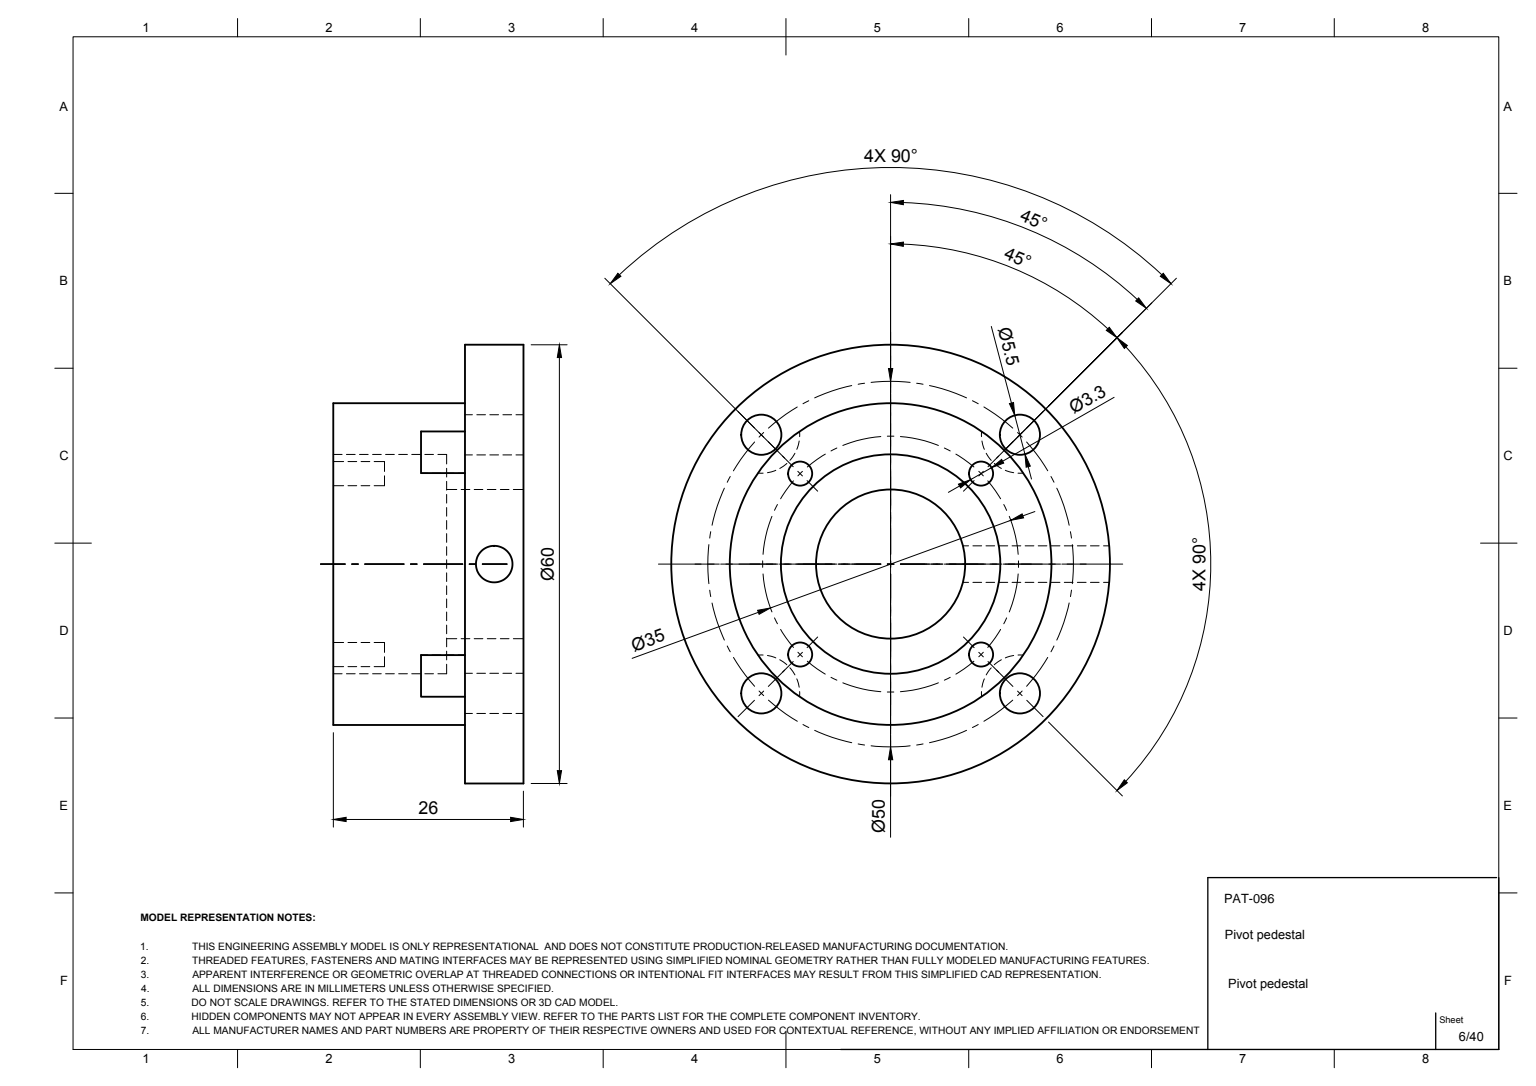
ISO-10303-21;
HEADER;
/* Generated by software containing ST-Developer
 * from STEP Tools, Inc. (www.steptools.com) 
 */

FILE_DESCRIPTION(
/* description */ ('PAT-096'),
/* implementation_level */ '2;1');

FILE_NAME(
/* name */ 'Pivot pedestal.step',
/* time_stamp */ '2026-10-29T17:03:14-07:00',
/* author */ (''),
/* organization */ (''),
/* preprocessor_version */ 'ST-DEVELOPER v20.2',
/* originating_system */ 'Autodesk Translation Framework v15.17.0.0',
/* authorisation */ '');

FILE_SCHEMA (('AUTOMOTIVE_DESIGN { 1 0 10303 214 3 1 1 }'));
ENDSEC;

DATA;
#10=MECHANICAL_DESIGN_GEOMETRIC_PRESENTATION_REPRESENTATION('',(#400),#10650);
#281=B_SPLINE_CURVE_WITH_KNOTS('',3,(#8659,#8660,#8661,#8662,#8663,#8664,
#8665,#8666,#8667,#8668),.UNSPECIFIED.,.F.,.F.,(4,2,2,2,4),(0.,0.0945941824764479,
0.189188364952896,0.283770357603024,0.378352350253152),.UNSPECIFIED.);
#282=B_SPLINE_CURVE_WITH_KNOTS('',3,(#8669,#8670,#8671,#8672,#8673,#8674,
#8675,#8676,#8677,#8678,#8679,#8680,#8681,#8682,#8683,#8684,#8685,#8686,
#8687,#8688,#8689,#8690,#8691,#8692,#8693,#8694),.UNSPECIFIED.,.F.,.F.,
(4,2,2,2,2,2,2,2,2,2,2,2,4),(0.378352350253152,0.47293434290328,0.567516335553408,
0.662110518029855,0.756704700506303,0.851298882982751,0.945893065459199,
1.04047505810933,1.13505705075946,1.22963904340958,1.32422103605971,1.41881521853616,
1.51340940101261),.UNSPECIFIED.);
#283=B_SPLINE_CURVE_WITH_KNOTS('',3,(#8698,#8699,#8700,#8701,#8702,#8703,
#8704,#8705,#8706,#8707,#8708,#8709,#8710,#8711,#8712,#8713,#8714,#8715,
#8716,#8717,#8718,#8719,#8720,#8721,#8722,#8723),.UNSPECIFIED.,.F.,.F.,
(4,2,2,2,2,2,2,2,2,2,2,2,4),(0.,0.0942186410044058,0.188437282008812,0.282655768798837,
0.376874255588861,0.471092742378886,0.565311229168911,0.659529870173317,
0.753748511177723,0.847967152182129,0.942185793186535,1.03640427997656,
1.13062276676658),.UNSPECIFIED.);
#284=B_SPLINE_CURVE_WITH_KNOTS('',3,(#8724,#8725,#8726,#8727,#8728,#8729,
#8730,#8731,#8732,#8733),.UNSPECIFIED.,.F.,.F.,(4,2,2,2,4),(1.13062276676658,
1.22484125355661,1.31905974034663,1.41327838135104,1.50749702235545),
 .UNSPECIFIED.);
#338=SHAPE_REPRESENTATION_RELATIONSHIP('SRR','None',#10798,#369);
#369=ADVANCED_BREP_SHAPE_REPRESENTATION('',(#438),#10616);
#400=STYLED_ITEM('',(#11078),#438);
#438=MANIFOLD_SOLID_BREP('Body1',#5534);
#490=FACE_BOUND('',#1192,.T.);
#491=FACE_BOUND('',#1193,.T.);
#492=FACE_BOUND('',#1194,.T.);
#493=FACE_BOUND('',#1195,.T.);
#494=FACE_BOUND('',#1196,.T.);
#495=FACE_BOUND('',#1203,.T.);
#496=FACE_BOUND('',#1205,.T.);
#497=FACE_BOUND('',#1207,.T.);
#498=FACE_BOUND('',#1209,.T.);
#499=FACE_BOUND('',#1210,.T.);
#500=FACE_BOUND('',#1211,.T.);
#501=FACE_BOUND('',#1212,.T.);
#502=FACE_BOUND('',#1213,.T.);
#503=FACE_BOUND('',#1215,.T.);
#504=FACE_BOUND('',#1216,.T.);
#505=FACE_BOUND('',#1217,.T.);
#506=FACE_BOUND('',#1218,.T.);
#507=FACE_BOUND('',#1219,.T.);
#629=PLANE('',#5977);
#630=PLANE('',#5981);
#631=PLANE('',#5985);
#632=PLANE('',#5989);
#633=PLANE('',#5990);
#634=PLANE('',#5998);
#635=PLANE('',#6003);
#636=PLANE('',#6008);
#637=PLANE('',#6017);
#638=PLANE('',#6034);
#639=PLANE('',#6040);
#640=PLANE('',#6041);
#820=FACE_OUTER_BOUND('',#1173,.T.);
#821=FACE_OUTER_BOUND('',#1174,.T.);
#822=FACE_OUTER_BOUND('',#1175,.T.);
#823=FACE_OUTER_BOUND('',#1176,.T.);
#824=FACE_OUTER_BOUND('',#1177,.T.);
#825=FACE_OUTER_BOUND('',#1178,.T.);
#826=FACE_OUTER_BOUND('',#1179,.T.);
#827=FACE_OUTER_BOUND('',#1180,.T.);
#828=FACE_OUTER_BOUND('',#1181,.T.);
#829=FACE_OUTER_BOUND('',#1182,.T.);
#830=FACE_OUTER_BOUND('',#1183,.T.);
#831=FACE_OUTER_BOUND('',#1184,.T.);
#832=FACE_OUTER_BOUND('',#1185,.T.);
#833=FACE_OUTER_BOUND('',#1186,.T.);
#834=FACE_OUTER_BOUND('',#1187,.T.);
#835=FACE_OUTER_BOUND('',#1188,.T.);
#836=FACE_OUTER_BOUND('',#1189,.T.);
#837=FACE_OUTER_BOUND('',#1190,.T.);
#838=FACE_OUTER_BOUND('',#1191,.T.);
#839=FACE_OUTER_BOUND('',#1197,.T.);
#840=FACE_OUTER_BOUND('',#1198,.T.);
#841=FACE_OUTER_BOUND('',#1199,.T.);
#842=FACE_OUTER_BOUND('',#1200,.T.);
#843=FACE_OUTER_BOUND('',#1201,.T.);
#844=FACE_OUTER_BOUND('',#1202,.T.);
#845=FACE_OUTER_BOUND('',#1204,.T.);
#846=FACE_OUTER_BOUND('',#1206,.T.);
#847=FACE_OUTER_BOUND('',#1208,.T.);
#848=FACE_OUTER_BOUND('',#1214,.T.);
#1173=EDGE_LOOP('',(#3847,#3848,#3849,#3850,#3851,#3852));
#1174=EDGE_LOOP('',(#3853,#3854,#3855,#3856));
#1175=EDGE_LOOP('',(#3857));
#1176=EDGE_LOOP('',(#3858,#3859,#3860,#3861));
#1177=EDGE_LOOP('',(#3862));
#1178=EDGE_LOOP('',(#3863,#3864,#3865,#3866));
#1179=EDGE_LOOP('',(#3867));
#1180=EDGE_LOOP('',(#3868,#3869,#3870,#3871));
#1181=EDGE_LOOP('',(#3872));
#1182=EDGE_LOOP('',(#3873,#3874));
#1183=EDGE_LOOP('',(#3875,#3876,#3877,#3878));
#1184=EDGE_LOOP('',(#3879,#3880,#3881,#3882));
#1185=EDGE_LOOP('',(#3883,#3884));
#1186=EDGE_LOOP('',(#3885,#3886,#3887,#3888));
#1187=EDGE_LOOP('',(#3889,#3890));
#1188=EDGE_LOOP('',(#3891,#3892,#3893,#3894));
#1189=EDGE_LOOP('',(#3895,#3896));
#1190=EDGE_LOOP('',(#3897,#3898,#3899,#3900,#3901,#3902,#3903,#3904,#3905,
#3906,#3907,#3908,#3909,#3910,#3911,#3912,#3913,#3914,#3915,#3916));
#1191=EDGE_LOOP('',(#3917));
#1192=EDGE_LOOP('',(#3918,#3919,#3920,#3921,#3922,#3923,#3924,#3925,#3926));
#1193=EDGE_LOOP('',(#3927));
#1194=EDGE_LOOP('',(#3928));
#1195=EDGE_LOOP('',(#3929));
#1196=EDGE_LOOP('',(#3930));
#1197=EDGE_LOOP('',(#3931,#3932,#3933,#3934));
#1198=EDGE_LOOP('',(#3935,#3936,#3937,#3938));
#1199=EDGE_LOOP('',(#3939,#3940,#3941,#3942));
#1200=EDGE_LOOP('',(#3943,#3944,#3945,#3946));
#1201=EDGE_LOOP('',(#3947,#3948,#3949,#3950));
#1202=EDGE_LOOP('',(#3951));
#1203=EDGE_LOOP('',(#3952));
#1204=EDGE_LOOP('',(#3953,#3954,#3955,#3956));
#1205=EDGE_LOOP('',(#3957,#3958));
#1206=EDGE_LOOP('',(#3959,#3960,#3961,#3962));
#1207=EDGE_LOOP('',(#3963,#3964));
#1208=EDGE_LOOP('',(#3965));
#1209=EDGE_LOOP('',(#3966));
#1210=EDGE_LOOP('',(#3967));
#1211=EDGE_LOOP('',(#3968));
#1212=EDGE_LOOP('',(#3969));
#1213=EDGE_LOOP('',(#3970));
#1214=EDGE_LOOP('',(#3971));
#1215=EDGE_LOOP('',(#3972));
#1216=EDGE_LOOP('',(#3973));
#1217=EDGE_LOOP('',(#3974));
#1218=EDGE_LOOP('',(#3975));
#1219=EDGE_LOOP('',(#3976));
#1644=LINE('',#8696,#1973);
#1645=LINE('',#8738,#1974);
#1646=LINE('',#8745,#1975);
#1647=LINE('',#8752,#1976);
#1648=LINE('',#8759,#1977);
#1649=LINE('',#8769,#1978);
#1650=LINE('',#8772,#1979);
#1651=LINE('',#8776,#1980);
#1652=LINE('',#8780,#1981);
#1653=LINE('',#8787,#1982);
#1654=LINE('',#8791,#1983);
#1655=LINE('',#8798,#1984);
#1656=LINE('',#8802,#1985);
#1657=LINE('',#8810,#1986);
#1658=LINE('',#8830,#1987);
#1659=LINE('',#8834,#1988);
#1660=LINE('',#8838,#1989);
#1661=LINE('',#8842,#1990);
#1662=LINE('',#8847,#1991);
#1663=LINE('',#8854,#1992);
#1664=LINE('',#8858,#1993);
#1973=VECTOR('',#6832,0.25);
#1974=VECTOR('',#6837,0.165);
#1975=VECTOR('',#6846,0.165);
#1976=VECTOR('',#6855,0.165);
#1977=VECTOR('',#6864,0.165);
#1978=VECTOR('',#6877,1.);
#1979=VECTOR('',#6880,1.);
#1980=VECTOR('',#6883,1.);
#1981=VECTOR('',#6886,1.);
#1982=VECTOR('',#6895,1.);
#1983=VECTOR('',#6898,1.);
#1984=VECTOR('',#6907,1.);
#1985=VECTOR('',#6910,1.);
#1986=VECTOR('',#6921,2.2);
#1987=VECTOR('',#6948,0.275);
#1988=VECTOR('',#6953,0.275);
#1989=VECTOR('',#6958,0.275);
#1990=VECTOR('',#6963,0.275);
#1991=VECTOR('',#6968,1.5);
#1992=VECTOR('',#6977,3.);
#1993=VECTOR('',#6982,1.02);
#2282=CIRCLE('',#5975,0.165);
#2283=CIRCLE('',#5976,0.165);
#2284=CIRCLE('',#5979,0.165);
#2285=CIRCLE('',#5980,0.165);
#2286=CIRCLE('',#5983,0.165);
#2287=CIRCLE('',#5984,0.165);
#2288=CIRCLE('',#5987,0.165);
#2289=CIRCLE('',#5988,0.165);
#2290=CIRCLE('',#5991,2.2);
#2291=CIRCLE('',#5992,0.525);
#2292=CIRCLE('',#5994,0.525);
#2293=CIRCLE('',#5996,0.525);
#2294=CIRCLE('',#5997,0.525);
#2295=CIRCLE('',#5999,2.2);
#2296=CIRCLE('',#6001,0.525);
#2297=CIRCLE('',#6002,0.525);
#2298=CIRCLE('',#6004,2.2);
#2299=CIRCLE('',#6006,0.525);
#2300=CIRCLE('',#6007,0.525);
#2301=CIRCLE('',#6009,2.2);
#2302=CIRCLE('',#6011,2.2);
#2303=CIRCLE('',#6012,2.2);
#2304=CIRCLE('',#6013,2.2);
#2305=CIRCLE('',#6014,2.2);
#2306=CIRCLE('',#6015,2.2);
#2307=CIRCLE('',#6016,2.2);
#2308=CIRCLE('',#6018,3.);
#2309=CIRCLE('',#6019,0.275);
#2310=CIRCLE('',#6020,0.275);
#2311=CIRCLE('',#6021,0.275);
#2312=CIRCLE('',#6022,0.275);
#2313=CIRCLE('',#6024,0.275);
#2314=CIRCLE('',#6026,0.275);
#2315=CIRCLE('',#6028,0.275);
#2316=CIRCLE('',#6030,0.275);
#2317=CIRCLE('',#6032,1.5);
#2318=CIRCLE('',#6033,1.5);
#2319=CIRCLE('',#6035,1.02);
#2320=CIRCLE('',#6037,3.);
#2321=CIRCLE('',#6039,1.02);
#2621=VERTEX_POINT('',#8657);
#2622=VERTEX_POINT('',#8658);
#2623=VERTEX_POINT('',#8695);
#2624=VERTEX_POINT('',#8697);
#2625=VERTEX_POINT('',#8735);
#2626=VERTEX_POINT('',#8737);
#2627=VERTEX_POINT('',#8742);
#2628=VERTEX_POINT('',#8744);
#2629=VERTEX_POINT('',#8749);
#2630=VERTEX_POINT('',#8751);
#2631=VERTEX_POINT('',#8756);
#2632=VERTEX_POINT('',#8758);
#2633=VERTEX_POINT('',#8763);
#2634=VERTEX_POINT('',#8764);
#2635=VERTEX_POINT('',#8768);
#2636=VERTEX_POINT('',#8770);
#2637=VERTEX_POINT('',#8774);
#2638=VERTEX_POINT('',#8775);
#2639=VERTEX_POINT('',#8777);
#2640=VERTEX_POINT('',#8779);
#2641=VERTEX_POINT('',#8785);
#2642=VERTEX_POINT('',#8786);
#2643=VERTEX_POINT('',#8788);
#2644=VERTEX_POINT('',#8790);
#2645=VERTEX_POINT('',#8796);
#2646=VERTEX_POINT('',#8797);
#2647=VERTEX_POINT('',#8799);
#2648=VERTEX_POINT('',#8801);
#2649=VERTEX_POINT('',#8807);
#2650=VERTEX_POINT('',#8809);
#2651=VERTEX_POINT('',#8817);
#2652=VERTEX_POINT('',#8819);
#2653=VERTEX_POINT('',#8821);
#2654=VERTEX_POINT('',#8823);
#2655=VERTEX_POINT('',#8825);
#2656=VERTEX_POINT('',#8828);
#2657=VERTEX_POINT('',#8832);
#2658=VERTEX_POINT('',#8836);
#2659=VERTEX_POINT('',#8840);
#2660=VERTEX_POINT('',#8844);
#2661=VERTEX_POINT('',#8846);
#2662=VERTEX_POINT('',#8850);
#2663=VERTEX_POINT('',#8853);
#2664=VERTEX_POINT('',#8857);
#3102=EDGE_CURVE('',#2621,#2622,#281,.T.);
#3103=EDGE_CURVE('',#2622,#2621,#282,.T.);
#3104=EDGE_CURVE('',#2622,#2623,#1644,.T.);
#3105=EDGE_CURVE('',#2624,#2623,#283,.T.);
#3106=EDGE_CURVE('',#2623,#2624,#284,.T.);
#3107=EDGE_CURVE('',#2625,#2625,#2282,.T.);
#3108=EDGE_CURVE('',#2625,#2626,#1645,.T.);
#3109=EDGE_CURVE('',#2626,#2626,#2283,.T.);
#3110=EDGE_CURVE('',#2627,#2627,#2284,.T.);
#3111=EDGE_CURVE('',#2627,#2628,#1646,.T.);
#3112=EDGE_CURVE('',#2628,#2628,#2285,.T.);
#3113=EDGE_CURVE('',#2629,#2629,#2286,.T.);
#3114=EDGE_CURVE('',#2629,#2630,#1647,.T.);
#3115=EDGE_CURVE('',#2630,#2630,#2287,.T.);
#3116=EDGE_CURVE('',#2631,#2631,#2288,.T.);
#3117=EDGE_CURVE('',#2631,#2632,#1648,.T.);
#3118=EDGE_CURVE('',#2632,#2632,#2289,.T.);
#3119=EDGE_CURVE('',#2633,#2634,#2290,.T.);
#3120=EDGE_CURVE('',#2634,#2633,#2291,.T.);
#3121=EDGE_CURVE('',#2635,#2633,#1649,.T.);
#3122=EDGE_CURVE('',#2636,#2635,#2292,.T.);
#3123=EDGE_CURVE('',#2634,#2636,#1650,.T.);
#3124=EDGE_CURVE('',#2637,#2638,#1651,.T.);
#3125=EDGE_CURVE('',#2637,#2639,#2293,.T.);
#3126=EDGE_CURVE('',#2640,#2639,#1652,.T.);
#3127=EDGE_CURVE('',#2638,#2640,#2294,.T.);
#3128=EDGE_CURVE('',#2639,#2637,#2295,.T.);
#3129=EDGE_CURVE('',#2641,#2642,#1653,.T.);
#3130=EDGE_CURVE('',#2641,#2643,#2296,.T.);
#3131=EDGE_CURVE('',#2644,#2643,#1654,.T.);
#3132=EDGE_CURVE('',#2642,#2644,#2297,.T.);
#3133=EDGE_CURVE('',#2643,#2641,#2298,.T.);
#3134=EDGE_CURVE('',#2645,#2646,#1655,.T.);
#3135=EDGE_CURVE('',#2645,#2647,#2299,.T.);
#3136=EDGE_CURVE('',#2648,#2647,#1656,.T.);
#3137=EDGE_CURVE('',#2646,#2648,#2300,.T.);
#3138=EDGE_CURVE('',#2647,#2645,#2301,.T.);
#3139=EDGE_CURVE('',#2649,#2649,#2302,.T.);
#3140=EDGE_CURVE('',#2649,#2650,#1657,.T.);
#3141=EDGE_CURVE('',#2650,#2635,#2303,.T.);
#3142=EDGE_CURVE('',#2636,#2648,#2304,.T.);
#3143=EDGE_CURVE('',#2646,#2644,#2305,.T.);
#3144=EDGE_CURVE('',#2642,#2640,#2306,.T.);
#3145=EDGE_CURVE('',#2638,#2650,#2307,.T.);
#3146=EDGE_CURVE('',#2651,#2651,#2308,.T.);
#3147=EDGE_CURVE('',#2652,#2652,#2309,.T.);
#3148=EDGE_CURVE('',#2653,#2653,#2310,.T.);
#3149=EDGE_CURVE('',#2654,#2654,#2311,.T.);
#3150=EDGE_CURVE('',#2655,#2655,#2312,.T.);
#3151=EDGE_CURVE('',#2656,#2656,#2313,.T.);
#3152=EDGE_CURVE('',#2656,#2652,#1658,.T.);
#3153=EDGE_CURVE('',#2657,#2657,#2314,.T.);
#3154=EDGE_CURVE('',#2657,#2655,#1659,.T.);
#3155=EDGE_CURVE('',#2658,#2658,#2315,.T.);
#3156=EDGE_CURVE('',#2658,#2653,#1660,.T.);
#3157=EDGE_CURVE('',#2659,#2659,#2316,.T.);
#3158=EDGE_CURVE('',#2659,#2654,#1661,.T.);
#3159=EDGE_CURVE('',#2660,#2660,#2317,.T.);
#3160=EDGE_CURVE('',#2660,#2661,#1662,.T.);
#3161=EDGE_CURVE('',#2661,#2661,#2318,.T.);
#3162=EDGE_CURVE('',#2662,#2662,#2319,.T.);
#3163=EDGE_CURVE('',#2651,#2663,#1663,.T.);
#3164=EDGE_CURVE('',#2663,#2663,#2320,.T.);
#3165=EDGE_CURVE('',#2662,#2664,#1664,.T.);
#3166=EDGE_CURVE('',#2664,#2664,#2321,.T.);
#3847=ORIENTED_EDGE('',*,*,#3102,.F.);
#3848=ORIENTED_EDGE('',*,*,#3103,.F.);
#3849=ORIENTED_EDGE('',*,*,#3104,.T.);
#3850=ORIENTED_EDGE('',*,*,#3105,.F.);
#3851=ORIENTED_EDGE('',*,*,#3106,.F.);
#3852=ORIENTED_EDGE('',*,*,#3104,.F.);
#3853=ORIENTED_EDGE('',*,*,#3107,.F.);
#3854=ORIENTED_EDGE('',*,*,#3108,.T.);
#3855=ORIENTED_EDGE('',*,*,#3109,.F.);
#3856=ORIENTED_EDGE('',*,*,#3108,.F.);
#3857=ORIENTED_EDGE('',*,*,#3107,.T.);
#3858=ORIENTED_EDGE('',*,*,#3110,.F.);
#3859=ORIENTED_EDGE('',*,*,#3111,.T.);
#3860=ORIENTED_EDGE('',*,*,#3112,.F.);
#3861=ORIENTED_EDGE('',*,*,#3111,.F.);
#3862=ORIENTED_EDGE('',*,*,#3110,.T.);
#3863=ORIENTED_EDGE('',*,*,#3113,.F.);
#3864=ORIENTED_EDGE('',*,*,#3114,.T.);
#3865=ORIENTED_EDGE('',*,*,#3115,.F.);
#3866=ORIENTED_EDGE('',*,*,#3114,.F.);
#3867=ORIENTED_EDGE('',*,*,#3113,.T.);
#3868=ORIENTED_EDGE('',*,*,#3116,.F.);
#3869=ORIENTED_EDGE('',*,*,#3117,.T.);
#3870=ORIENTED_EDGE('',*,*,#3118,.F.);
#3871=ORIENTED_EDGE('',*,*,#3117,.F.);
#3872=ORIENTED_EDGE('',*,*,#3116,.T.);
#3873=ORIENTED_EDGE('',*,*,#3119,.F.);
#3874=ORIENTED_EDGE('',*,*,#3120,.F.);
#3875=ORIENTED_EDGE('',*,*,#3121,.F.);
#3876=ORIENTED_EDGE('',*,*,#3122,.F.);
#3877=ORIENTED_EDGE('',*,*,#3123,.F.);
#3878=ORIENTED_EDGE('',*,*,#3120,.T.);
#3879=ORIENTED_EDGE('',*,*,#3124,.F.);
#3880=ORIENTED_EDGE('',*,*,#3125,.T.);
#3881=ORIENTED_EDGE('',*,*,#3126,.F.);
#3882=ORIENTED_EDGE('',*,*,#3127,.F.);
#3883=ORIENTED_EDGE('',*,*,#3128,.F.);
#3884=ORIENTED_EDGE('',*,*,#3125,.F.);
#3885=ORIENTED_EDGE('',*,*,#3129,.F.);
#3886=ORIENTED_EDGE('',*,*,#3130,.T.);
#3887=ORIENTED_EDGE('',*,*,#3131,.F.);
#3888=ORIENTED_EDGE('',*,*,#3132,.F.);
#3889=ORIENTED_EDGE('',*,*,#3133,.F.);
#3890=ORIENTED_EDGE('',*,*,#3130,.F.);
#3891=ORIENTED_EDGE('',*,*,#3134,.F.);
#3892=ORIENTED_EDGE('',*,*,#3135,.T.);
#3893=ORIENTED_EDGE('',*,*,#3136,.F.);
#3894=ORIENTED_EDGE('',*,*,#3137,.F.);
#3895=ORIENTED_EDGE('',*,*,#3138,.F.);
#3896=ORIENTED_EDGE('',*,*,#3135,.F.);
#3897=ORIENTED_EDGE('',*,*,#3139,.F.);
#3898=ORIENTED_EDGE('',*,*,#3140,.T.);
#3899=ORIENTED_EDGE('',*,*,#3141,.T.);
#3900=ORIENTED_EDGE('',*,*,#3121,.T.);
#3901=ORIENTED_EDGE('',*,*,#3119,.T.);
#3902=ORIENTED_EDGE('',*,*,#3123,.T.);
#3903=ORIENTED_EDGE('',*,*,#3142,.T.);
#3904=ORIENTED_EDGE('',*,*,#3136,.T.);
#3905=ORIENTED_EDGE('',*,*,#3138,.T.);
#3906=ORIENTED_EDGE('',*,*,#3134,.T.);
#3907=ORIENTED_EDGE('',*,*,#3143,.T.);
#3908=ORIENTED_EDGE('',*,*,#3131,.T.);
#3909=ORIENTED_EDGE('',*,*,#3133,.T.);
#3910=ORIENTED_EDGE('',*,*,#3129,.T.);
#3911=ORIENTED_EDGE('',*,*,#3144,.T.);
#3912=ORIENTED_EDGE('',*,*,#3126,.T.);
#3913=ORIENTED_EDGE('',*,*,#3128,.T.);
#3914=ORIENTED_EDGE('',*,*,#3124,.T.);
#3915=ORIENTED_EDGE('',*,*,#3145,.T.);
#3916=ORIENTED_EDGE('',*,*,#3140,.F.);
#3917=ORIENTED_EDGE('',*,*,#3146,.T.);
#3918=ORIENTED_EDGE('',*,*,#3145,.F.);
#3919=ORIENTED_EDGE('',*,*,#3127,.T.);
#3920=ORIENTED_EDGE('',*,*,#3144,.F.);
#3921=ORIENTED_EDGE('',*,*,#3132,.T.);
#3922=ORIENTED_EDGE('',*,*,#3143,.F.);
#3923=ORIENTED_EDGE('',*,*,#3137,.T.);
#3924=ORIENTED_EDGE('',*,*,#3142,.F.);
#3925=ORIENTED_EDGE('',*,*,#3122,.T.);
#3926=ORIENTED_EDGE('',*,*,#3141,.F.);
#3927=ORIENTED_EDGE('',*,*,#3147,.T.);
#3928=ORIENTED_EDGE('',*,*,#3148,.T.);
#3929=ORIENTED_EDGE('',*,*,#3149,.T.);
#3930=ORIENTED_EDGE('',*,*,#3150,.T.);
#3931=ORIENTED_EDGE('',*,*,#3151,.F.);
#3932=ORIENTED_EDGE('',*,*,#3152,.T.);
#3933=ORIENTED_EDGE('',*,*,#3147,.F.);
#3934=ORIENTED_EDGE('',*,*,#3152,.F.);
#3935=ORIENTED_EDGE('',*,*,#3153,.F.);
#3936=ORIENTED_EDGE('',*,*,#3154,.T.);
#3937=ORIENTED_EDGE('',*,*,#3150,.F.);
#3938=ORIENTED_EDGE('',*,*,#3154,.F.);
#3939=ORIENTED_EDGE('',*,*,#3155,.F.);
#3940=ORIENTED_EDGE('',*,*,#3156,.T.);
#3941=ORIENTED_EDGE('',*,*,#3148,.F.);
#3942=ORIENTED_EDGE('',*,*,#3156,.F.);
#3943=ORIENTED_EDGE('',*,*,#3157,.F.);
#3944=ORIENTED_EDGE('',*,*,#3158,.T.);
#3945=ORIENTED_EDGE('',*,*,#3149,.F.);
#3946=ORIENTED_EDGE('',*,*,#3158,.F.);
#3947=ORIENTED_EDGE('',*,*,#3159,.F.);
#3948=ORIENTED_EDGE('',*,*,#3160,.T.);
#3949=ORIENTED_EDGE('',*,*,#3161,.F.);
#3950=ORIENTED_EDGE('',*,*,#3160,.F.);
#3951=ORIENTED_EDGE('',*,*,#3159,.T.);
#3952=ORIENTED_EDGE('',*,*,#3162,.F.);
#3953=ORIENTED_EDGE('',*,*,#3146,.F.);
#3954=ORIENTED_EDGE('',*,*,#3163,.T.);
#3955=ORIENTED_EDGE('',*,*,#3164,.T.);
#3956=ORIENTED_EDGE('',*,*,#3163,.F.);
#3957=ORIENTED_EDGE('',*,*,#3105,.T.);
#3958=ORIENTED_EDGE('',*,*,#3106,.T.);
#3959=ORIENTED_EDGE('',*,*,#3162,.T.);
#3960=ORIENTED_EDGE('',*,*,#3165,.T.);
#3961=ORIENTED_EDGE('',*,*,#3166,.T.);
#3962=ORIENTED_EDGE('',*,*,#3165,.F.);
#3963=ORIENTED_EDGE('',*,*,#3102,.T.);
#3964=ORIENTED_EDGE('',*,*,#3103,.T.);
#3965=ORIENTED_EDGE('',*,*,#3139,.T.);
#3966=ORIENTED_EDGE('',*,*,#3161,.T.);
#3967=ORIENTED_EDGE('',*,*,#3118,.T.);
#3968=ORIENTED_EDGE('',*,*,#3115,.T.);
#3969=ORIENTED_EDGE('',*,*,#3112,.T.);
#3970=ORIENTED_EDGE('',*,*,#3109,.T.);
#3971=ORIENTED_EDGE('',*,*,#3164,.F.);
#3972=ORIENTED_EDGE('',*,*,#3166,.F.);
#3973=ORIENTED_EDGE('',*,*,#3157,.T.);
#3974=ORIENTED_EDGE('',*,*,#3155,.T.);
#3975=ORIENTED_EDGE('',*,*,#3153,.T.);
#3976=ORIENTED_EDGE('',*,*,#3151,.T.);
#5083=CYLINDRICAL_SURFACE('',#5973,0.25);
#5084=CYLINDRICAL_SURFACE('',#5974,0.165);
#5085=CYLINDRICAL_SURFACE('',#5978,0.165);
#5086=CYLINDRICAL_SURFACE('',#5982,0.165);
#5087=CYLINDRICAL_SURFACE('',#5986,0.165);
#5088=CYLINDRICAL_SURFACE('',#5993,0.525);
#5089=CYLINDRICAL_SURFACE('',#5995,0.525);
#5090=CYLINDRICAL_SURFACE('',#6000,0.525);
#5091=CYLINDRICAL_SURFACE('',#6005,0.525);
#5092=CYLINDRICAL_SURFACE('',#6010,2.2);
#5093=CYLINDRICAL_SURFACE('',#6023,0.275);
#5094=CYLINDRICAL_SURFACE('',#6025,0.275);
#5095=CYLINDRICAL_SURFACE('',#6027,0.275);
#5096=CYLINDRICAL_SURFACE('',#6029,0.275);
#5097=CYLINDRICAL_SURFACE('',#6031,1.5);
#5098=CYLINDRICAL_SURFACE('',#6036,3.);
#5099=CYLINDRICAL_SURFACE('',#6038,1.02);
#5225=ADVANCED_FACE('',(#820),#5083,.F.);
#5226=ADVANCED_FACE('',(#821),#5084,.F.);
#5227=ADVANCED_FACE('',(#822),#629,.T.);
#5228=ADVANCED_FACE('',(#823),#5085,.F.);
#5229=ADVANCED_FACE('',(#824),#630,.T.);
#5230=ADVANCED_FACE('',(#825),#5086,.F.);
#5231=ADVANCED_FACE('',(#826),#631,.T.);
#5232=ADVANCED_FACE('',(#827),#5087,.F.);
#5233=ADVANCED_FACE('',(#828),#632,.T.);
#5234=ADVANCED_FACE('',(#829),#633,.F.);
#5235=ADVANCED_FACE('',(#830),#5088,.F.);
#5236=ADVANCED_FACE('',(#831),#5089,.F.);
#5237=ADVANCED_FACE('',(#832),#634,.F.);
#5238=ADVANCED_FACE('',(#833),#5090,.F.);
#5239=ADVANCED_FACE('',(#834),#635,.F.);
#5240=ADVANCED_FACE('',(#835),#5091,.F.);
#5241=ADVANCED_FACE('',(#836),#636,.F.);
#5242=ADVANCED_FACE('',(#837),#5092,.T.);
#5243=ADVANCED_FACE('',(#838,#490,#491,#492,#493,#494),#637,.T.);
#5244=ADVANCED_FACE('',(#839),#5093,.F.);
#5245=ADVANCED_FACE('',(#840),#5094,.F.);
#5246=ADVANCED_FACE('',(#841),#5095,.F.);
#5247=ADVANCED_FACE('',(#842),#5096,.F.);
#5248=ADVANCED_FACE('',(#843),#5097,.F.);
#5249=ADVANCED_FACE('',(#844,#495),#638,.T.);
#5250=ADVANCED_FACE('',(#845,#496),#5098,.T.);
#5251=ADVANCED_FACE('',(#846,#497),#5099,.F.);
#5252=ADVANCED_FACE('',(#847,#498,#499,#500,#501,#502),#639,.T.);
#5253=ADVANCED_FACE('',(#848,#503,#504,#505,#506,#507),#640,.F.);
#5534=CLOSED_SHELL('',(#5225,#5226,#5227,#5228,#5229,#5230,#5231,#5232,
#5233,#5234,#5235,#5236,#5237,#5238,#5239,#5240,#5241,#5242,#5243,#5244,
#5245,#5246,#5247,#5248,#5249,#5250,#5251,#5252,#5253));
#5972=AXIS2_PLACEMENT_3D('',#8655,#6828,#6829);
#5973=AXIS2_PLACEMENT_3D('',#8656,#6830,#6831);
#5974=AXIS2_PLACEMENT_3D('',#8734,#6833,#6834);
#5975=AXIS2_PLACEMENT_3D('',#8736,#6835,#6836);
#5976=AXIS2_PLACEMENT_3D('',#8739,#6838,#6839);
#5977=AXIS2_PLACEMENT_3D('',#8740,#6840,#6841);
#5978=AXIS2_PLACEMENT_3D('',#8741,#6842,#6843);
#5979=AXIS2_PLACEMENT_3D('',#8743,#6844,#6845);
#5980=AXIS2_PLACEMENT_3D('',#8746,#6847,#6848);
#5981=AXIS2_PLACEMENT_3D('',#8747,#6849,#6850);
#5982=AXIS2_PLACEMENT_3D('',#8748,#6851,#6852);
#5983=AXIS2_PLACEMENT_3D('',#8750,#6853,#6854);
#5984=AXIS2_PLACEMENT_3D('',#8753,#6856,#6857);
#5985=AXIS2_PLACEMENT_3D('',#8754,#6858,#6859);
#5986=AXIS2_PLACEMENT_3D('',#8755,#6860,#6861);
#5987=AXIS2_PLACEMENT_3D('',#8757,#6862,#6863);
#5988=AXIS2_PLACEMENT_3D('',#8760,#6865,#6866);
#5989=AXIS2_PLACEMENT_3D('',#8761,#6867,#6868);
#5990=AXIS2_PLACEMENT_3D('',#8762,#6869,#6870);
#5991=AXIS2_PLACEMENT_3D('',#8765,#6871,#6872);
#5992=AXIS2_PLACEMENT_3D('',#8766,#6873,#6874);
#5993=AXIS2_PLACEMENT_3D('',#8767,#6875,#6876);
#5994=AXIS2_PLACEMENT_3D('',#8771,#6878,#6879);
#5995=AXIS2_PLACEMENT_3D('',#8773,#6881,#6882);
#5996=AXIS2_PLACEMENT_3D('',#8778,#6884,#6885);
#5997=AXIS2_PLACEMENT_3D('',#8781,#6887,#6888);
#5998=AXIS2_PLACEMENT_3D('',#8782,#6889,#6890);
#5999=AXIS2_PLACEMENT_3D('',#8783,#6891,#6892);
#6000=AXIS2_PLACEMENT_3D('',#8784,#6893,#6894);
#6001=AXIS2_PLACEMENT_3D('',#8789,#6896,#6897);
#6002=AXIS2_PLACEMENT_3D('',#8792,#6899,#6900);
#6003=AXIS2_PLACEMENT_3D('',#8793,#6901,#6902);
#6004=AXIS2_PLACEMENT_3D('',#8794,#6903,#6904);
#6005=AXIS2_PLACEMENT_3D('',#8795,#6905,#6906);
#6006=AXIS2_PLACEMENT_3D('',#8800,#6908,#6909);
#6007=AXIS2_PLACEMENT_3D('',#8803,#6911,#6912);
#6008=AXIS2_PLACEMENT_3D('',#8804,#6913,#6914);
#6009=AXIS2_PLACEMENT_3D('',#8805,#6915,#6916);
#6010=AXIS2_PLACEMENT_3D('',#8806,#6917,#6918);
#6011=AXIS2_PLACEMENT_3D('',#8808,#6919,#6920);
#6012=AXIS2_PLACEMENT_3D('',#8811,#6922,#6923);
#6013=AXIS2_PLACEMENT_3D('',#8812,#6924,#6925);
#6014=AXIS2_PLACEMENT_3D('',#8813,#6926,#6927);
#6015=AXIS2_PLACEMENT_3D('',#8814,#6928,#6929);
#6016=AXIS2_PLACEMENT_3D('',#8815,#6930,#6931);
#6017=AXIS2_PLACEMENT_3D('',#8816,#6932,#6933);
#6018=AXIS2_PLACEMENT_3D('',#8818,#6934,#6935);
#6019=AXIS2_PLACEMENT_3D('',#8820,#6936,#6937);
#6020=AXIS2_PLACEMENT_3D('',#8822,#6938,#6939);
#6021=AXIS2_PLACEMENT_3D('',#8824,#6940,#6941);
#6022=AXIS2_PLACEMENT_3D('',#8826,#6942,#6943);
#6023=AXIS2_PLACEMENT_3D('',#8827,#6944,#6945);
#6024=AXIS2_PLACEMENT_3D('',#8829,#6946,#6947);
#6025=AXIS2_PLACEMENT_3D('',#8831,#6949,#6950);
#6026=AXIS2_PLACEMENT_3D('',#8833,#6951,#6952);
#6027=AXIS2_PLACEMENT_3D('',#8835,#6954,#6955);
#6028=AXIS2_PLACEMENT_3D('',#8837,#6956,#6957);
#6029=AXIS2_PLACEMENT_3D('',#8839,#6959,#6960);
#6030=AXIS2_PLACEMENT_3D('',#8841,#6961,#6962);
#6031=AXIS2_PLACEMENT_3D('',#8843,#6964,#6965);
#6032=AXIS2_PLACEMENT_3D('',#8845,#6966,#6967);
#6033=AXIS2_PLACEMENT_3D('',#8848,#6969,#6970);
#6034=AXIS2_PLACEMENT_3D('',#8849,#6971,#6972);
#6035=AXIS2_PLACEMENT_3D('',#8851,#6973,#6974);
#6036=AXIS2_PLACEMENT_3D('',#8852,#6975,#6976);
#6037=AXIS2_PLACEMENT_3D('',#8855,#6978,#6979);
#6038=AXIS2_PLACEMENT_3D('',#8856,#6980,#6981);
#6039=AXIS2_PLACEMENT_3D('',#8859,#6983,#6984);
#6040=AXIS2_PLACEMENT_3D('',#8860,#6985,#6986);
#6041=AXIS2_PLACEMENT_3D('',#8861,#6987,#6988);
#6828=DIRECTION('axis',(0.,0.,1.));
#6829=DIRECTION('refdir',(1.,0.,0.));
#6830=DIRECTION('center_axis',(1.,0.,0.));
#6831=DIRECTION('ref_axis',(0.,0.,-1.));
#6832=DIRECTION('',(1.,0.,0.));
#6833=DIRECTION('center_axis',(0.,0.,1.));
#6834=DIRECTION('ref_axis',(1.,0.,0.));
#6835=DIRECTION('center_axis',(0.,0.,1.));
#6836=DIRECTION('ref_axis',(1.,0.,0.));
#6837=DIRECTION('',(0.,0.,1.));
#6838=DIRECTION('center_axis',(0.,0.,-1.));
#6839=DIRECTION('ref_axis',(1.,0.,0.));
#6840=DIRECTION('center_axis',(0.,0.,1.));
#6841=DIRECTION('ref_axis',(1.,0.,0.));
#6842=DIRECTION('center_axis',(0.,0.,1.));
#6843=DIRECTION('ref_axis',(1.,0.,0.));
#6844=DIRECTION('center_axis',(0.,0.,1.));
#6845=DIRECTION('ref_axis',(1.,0.,0.));
#6846=DIRECTION('',(0.,0.,1.));
#6847=DIRECTION('center_axis',(0.,0.,-1.));
#6848=DIRECTION('ref_axis',(1.,0.,0.));
#6849=DIRECTION('center_axis',(0.,0.,1.));
#6850=DIRECTION('ref_axis',(1.,0.,0.));
#6851=DIRECTION('center_axis',(0.,0.,1.));
#6852=DIRECTION('ref_axis',(1.,0.,0.));
#6853=DIRECTION('center_axis',(0.,0.,1.));
#6854=DIRECTION('ref_axis',(1.,0.,0.));
#6855=DIRECTION('',(0.,0.,1.));
#6856=DIRECTION('center_axis',(0.,0.,-1.));
#6857=DIRECTION('ref_axis',(1.,0.,0.));
#6858=DIRECTION('center_axis',(0.,0.,1.));
#6859=DIRECTION('ref_axis',(1.,0.,0.));
#6860=DIRECTION('center_axis',(0.,0.,1.));
#6861=DIRECTION('ref_axis',(1.,0.,0.));
#6862=DIRECTION('center_axis',(0.,0.,1.));
#6863=DIRECTION('ref_axis',(1.,0.,0.));
#6864=DIRECTION('',(0.,0.,1.));
#6865=DIRECTION('center_axis',(0.,0.,-1.));
#6866=DIRECTION('ref_axis',(1.,0.,0.));
#6867=DIRECTION('center_axis',(0.,0.,1.));
#6868=DIRECTION('ref_axis',(1.,0.,0.));
#6869=DIRECTION('center_axis',(0.,0.,1.));
#6870=DIRECTION('ref_axis',(1.,0.,0.));
#6871=DIRECTION('center_axis',(0.,0.,1.));
#6872=DIRECTION('ref_axis',(1.,0.,0.));
#6873=DIRECTION('center_axis',(0.,0.,1.));
#6874=DIRECTION('ref_axis',(1.,0.,0.));
#6875=DIRECTION('center_axis',(0.,0.,1.));
#6876=DIRECTION('ref_axis',(1.,0.,0.));
#6877=DIRECTION('',(0.,0.,1.));
#6878=DIRECTION('center_axis',(0.,0.,1.));
#6879=DIRECTION('ref_axis',(1.,0.,0.));
#6880=DIRECTION('',(0.,0.,-1.));
#6881=DIRECTION('center_axis',(0.,0.,1.));
#6882=DIRECTION('ref_axis',(1.,0.,0.));
#6883=DIRECTION('',(0.,0.,-1.));
#6884=DIRECTION('center_axis',(0.,0.,1.));
#6885=DIRECTION('ref_axis',(1.,0.,0.));
#6886=DIRECTION('',(0.,0.,1.));
#6887=DIRECTION('center_axis',(0.,0.,1.));
#6888=DIRECTION('ref_axis',(1.,0.,0.));
#6889=DIRECTION('center_axis',(0.,0.,1.));
#6890=DIRECTION('ref_axis',(1.,0.,0.));
#6891=DIRECTION('center_axis',(0.,0.,1.));
#6892=DIRECTION('ref_axis',(1.,0.,0.));
#6893=DIRECTION('center_axis',(0.,0.,1.));
#6894=DIRECTION('ref_axis',(-0.707106781186548,-0.707106781186547,0.));
#6895=DIRECTION('',(0.,0.,-1.));
#6896=DIRECTION('center_axis',(0.,0.,1.));
#6897=DIRECTION('ref_axis',(1.,0.,0.));
#6898=DIRECTION('',(0.,0.,1.));
#6899=DIRECTION('center_axis',(0.,0.,1.));
#6900=DIRECTION('ref_axis',(1.,0.,0.));
#6901=DIRECTION('center_axis',(0.,0.,1.));
#6902=DIRECTION('ref_axis',(1.,0.,0.));
#6903=DIRECTION('center_axis',(0.,0.,1.));
#6904=DIRECTION('ref_axis',(1.,0.,0.));
#6905=DIRECTION('center_axis',(0.,0.,1.));
#6906=DIRECTION('ref_axis',(-0.707106781186547,0.707106781186548,0.));
#6907=DIRECTION('',(0.,0.,-1.));
#6908=DIRECTION('center_axis',(0.,0.,1.));
#6909=DIRECTION('ref_axis',(1.,0.,0.));
#6910=DIRECTION('',(0.,0.,1.));
#6911=DIRECTION('center_axis',(0.,0.,1.));
#6912=DIRECTION('ref_axis',(1.,0.,0.));
#6913=DIRECTION('center_axis',(0.,0.,1.));
#6914=DIRECTION('ref_axis',(1.,0.,0.));
#6915=DIRECTION('center_axis',(0.,0.,1.));
#6916=DIRECTION('ref_axis',(1.,0.,0.));
#6917=DIRECTION('center_axis',(0.,0.,1.));
#6918=DIRECTION('ref_axis',(1.,0.,0.));
#6919=DIRECTION('center_axis',(0.,0.,1.));
#6920=DIRECTION('ref_axis',(1.,0.,0.));
#6921=DIRECTION('',(0.,0.,-1.));
#6922=DIRECTION('center_axis',(0.,0.,1.));
#6923=DIRECTION('ref_axis',(1.,0.,0.));
#6924=DIRECTION('center_axis',(0.,0.,1.));
#6925=DIRECTION('ref_axis',(1.,0.,0.));
#6926=DIRECTION('center_axis',(0.,0.,1.));
#6927=DIRECTION('ref_axis',(1.,0.,0.));
#6928=DIRECTION('center_axis',(0.,0.,1.));
#6929=DIRECTION('ref_axis',(1.,0.,0.));
#6930=DIRECTION('center_axis',(0.,0.,1.));
#6931=DIRECTION('ref_axis',(1.,0.,0.));
#6932=DIRECTION('center_axis',(0.,0.,1.));
#6933=DIRECTION('ref_axis',(1.,0.,0.));
#6934=DIRECTION('center_axis',(0.,0.,1.));
#6935=DIRECTION('ref_axis',(1.,0.,0.));
#6936=DIRECTION('center_axis',(0.,0.,-1.));
#6937=DIRECTION('ref_axis',(1.,0.,0.));
#6938=DIRECTION('center_axis',(0.,0.,-1.));
#6939=DIRECTION('ref_axis',(1.,0.,0.));
#6940=DIRECTION('center_axis',(0.,0.,-1.));
#6941=DIRECTION('ref_axis',(1.,0.,0.));
#6942=DIRECTION('center_axis',(0.,0.,-1.));
#6943=DIRECTION('ref_axis',(1.,0.,0.));
#6944=DIRECTION('center_axis',(0.,0.,1.));
#6945=DIRECTION('ref_axis',(1.,0.,0.));
#6946=DIRECTION('center_axis',(0.,0.,1.));
#6947=DIRECTION('ref_axis',(1.,0.,0.));
#6948=DIRECTION('',(0.,0.,1.));
#6949=DIRECTION('center_axis',(0.,0.,1.));
#6950=DIRECTION('ref_axis',(1.,0.,0.));
#6951=DIRECTION('center_axis',(0.,0.,1.));
#6952=DIRECTION('ref_axis',(1.,0.,0.));
#6953=DIRECTION('',(0.,0.,1.));
#6954=DIRECTION('center_axis',(0.,0.,1.));
#6955=DIRECTION('ref_axis',(1.,0.,0.));
#6956=DIRECTION('center_axis',(0.,0.,1.));
#6957=DIRECTION('ref_axis',(1.,0.,0.));
#6958=DIRECTION('',(0.,0.,1.));
#6959=DIRECTION('center_axis',(0.,0.,1.));
#6960=DIRECTION('ref_axis',(1.,0.,0.));
#6961=DIRECTION('center_axis',(0.,0.,1.));
#6962=DIRECTION('ref_axis',(1.,0.,0.));
#6963=DIRECTION('',(0.,0.,1.));
#6964=DIRECTION('center_axis',(0.,0.,1.));
#6965=DIRECTION('ref_axis',(1.,0.,0.));
#6966=DIRECTION('center_axis',(0.,0.,1.));
#6967=DIRECTION('ref_axis',(1.,0.,0.));
#6968=DIRECTION('',(0.,0.,1.));
#6969=DIRECTION('center_axis',(0.,0.,-1.));
#6970=DIRECTION('ref_axis',(1.,0.,0.));
#6971=DIRECTION('center_axis',(0.,0.,1.));
#6972=DIRECTION('ref_axis',(1.,0.,0.));
#6973=DIRECTION('center_axis',(0.,0.,1.));
#6974=DIRECTION('ref_axis',(1.,0.,0.));
#6975=DIRECTION('center_axis',(0.,0.,1.));
#6976=DIRECTION('ref_axis',(1.,0.,0.));
#6977=DIRECTION('',(0.,0.,-1.));
#6978=DIRECTION('center_axis',(0.,0.,1.));
#6979=DIRECTION('ref_axis',(1.,0.,0.));
#6980=DIRECTION('center_axis',(0.,0.,1.));
#6981=DIRECTION('ref_axis',(1.,0.,0.));
#6982=DIRECTION('',(0.,0.,-1.));
#6983=DIRECTION('center_axis',(0.,0.,-1.));
#6984=DIRECTION('ref_axis',(1.,0.,0.));
#6985=DIRECTION('center_axis',(0.,0.,1.));
#6986=DIRECTION('ref_axis',(1.,0.,0.));
#6987=DIRECTION('center_axis',(0.,0.,1.));
#6988=DIRECTION('ref_axis',(1.,0.,0.));
#8655=CARTESIAN_POINT('',(0.,0.,0.));
#8656=CARTESIAN_POINT('Origin',(0.9,0.,1.4));
#8657=CARTESIAN_POINT('',(0.988888264668966,0.25,1.4));
#8658=CARTESIAN_POINT('',(1.02,-1.18386380373883E-17,1.65));
#8659=CARTESIAN_POINT('Ctrl Pts',(0.988888264668966,0.25,1.4));
#8660=CARTESIAN_POINT('Ctrl Pts',(0.988888264668966,0.25,1.43153139415882));
#8661=CARTESIAN_POINT('Ctrl Pts',(0.990553370646674,0.243672048431404,1.46507214966317));
#8662=CARTESIAN_POINT('Ctrl Pts',(0.996491737296663,0.218119830014375,1.52662620974954));
#8663=CARTESIAN_POINT('Ctrl Pts',(1.00067109353237,0.198902128206072,1.5546512623872));
#8664=CARTESIAN_POINT('Ctrl Pts',(1.00845756932386,0.154654113568716,1.59889927702456));
#8665=CARTESIAN_POINT('Ctrl Pts',(1.01258144235289,0.126627870945253,1.61811920309393));
#8666=CARTESIAN_POINT('Ctrl Pts',(1.0183917429657,0.065069600391363,1.64367304400768));
#8667=CARTESIAN_POINT('Ctrl Pts',(1.02,0.031527330883376,1.65));
#8668=CARTESIAN_POINT('Ctrl Pts',(1.02,2.77555756156289E-17,1.65));
#8669=CARTESIAN_POINT('Ctrl Pts',(1.02,6.93889390390723E-18,1.65));
#8670=CARTESIAN_POINT('Ctrl Pts',(1.02,-0.031527330883376,1.65));
#8671=CARTESIAN_POINT('Ctrl Pts',(1.0183917429657,-0.065069600391363,1.64367304400768));
#8672=CARTESIAN_POINT('Ctrl Pts',(1.01258144235289,-0.126627870945253,1.61811920309393));
#8673=CARTESIAN_POINT('Ctrl Pts',(1.00845756932386,-0.154654113568716,1.59889927702456));
#8674=CARTESIAN_POINT('Ctrl Pts',(1.00067109353237,-0.198902128206072,1.5546512623872));
#8675=CARTESIAN_POINT('Ctrl Pts',(0.996491737296663,-0.218119830014375,
1.52662620974954));
#8676=CARTESIAN_POINT('Ctrl Pts',(0.990553370646674,-0.243672048431404,
1.46507214966317));
#8677=CARTESIAN_POINT('Ctrl Pts',(0.988888264668967,-0.25,1.43153139415882));
#8678=CARTESIAN_POINT('Ctrl Pts',(0.988888264668967,-0.25,1.36846860584118));
#8679=CARTESIAN_POINT('Ctrl Pts',(0.990553370646674,-0.243672048431404,
1.33492785033683));
#8680=CARTESIAN_POINT('Ctrl Pts',(0.996491737296663,-0.218119830014375,
1.27337379025046));
#8681=CARTESIAN_POINT('Ctrl Pts',(1.00067109353237,-0.198902128206072,1.2453487376128));
#8682=CARTESIAN_POINT('Ctrl Pts',(1.00845756932386,-0.154654113568716,1.20110072297544));
#8683=CARTESIAN_POINT('Ctrl Pts',(1.01258144235289,-0.126627870945254,1.18188079690607));
#8684=CARTESIAN_POINT('Ctrl Pts',(1.0183917429657,-0.0650696003913633,1.15632695599232));
#8685=CARTESIAN_POINT('Ctrl Pts',(1.02,-0.0315273308833761,1.15));
#8686=CARTESIAN_POINT('Ctrl Pts',(1.02,0.0315273308833759,1.15));
#8687=CARTESIAN_POINT('Ctrl Pts',(1.0183917429657,0.065069600391363,1.15632695599232));
#8688=CARTESIAN_POINT('Ctrl Pts',(1.01258144235289,0.126627870945253,1.18188079690607));
#8689=CARTESIAN_POINT('Ctrl Pts',(1.00845756932386,0.154654113568716,1.20110072297544));
#8690=CARTESIAN_POINT('Ctrl Pts',(1.00067109353237,0.198902128206072,1.2453487376128));
#8691=CARTESIAN_POINT('Ctrl Pts',(0.996491737296663,0.218119830014375,1.27337379025046));
#8692=CARTESIAN_POINT('Ctrl Pts',(0.990553370646674,0.243672048431404,1.33492785033683));
#8693=CARTESIAN_POINT('Ctrl Pts',(0.988888264668967,0.25,1.36846860584118));
#8694=CARTESIAN_POINT('Ctrl Pts',(0.988888264668967,0.25,1.4));
#8695=CARTESIAN_POINT('',(3.,-3.06161699786838E-17,1.65));
#8696=CARTESIAN_POINT('',(0.9,-3.06161699786838E-17,1.65));
#8697=CARTESIAN_POINT('',(2.98956518577535,0.25,1.4));
#8698=CARTESIAN_POINT('Ctrl Pts',(2.98956518577535,0.25,1.4));
#8699=CARTESIAN_POINT('Ctrl Pts',(2.98956518577535,0.25,1.36859378633186));
#8700=CARTESIAN_POINT('Ctrl Pts',(2.99011104995181,0.24372047740942,1.33510417960069));
#8701=CARTESIAN_POINT('Ctrl Pts',(2.99208145165098,0.218202539734559,1.27351367328886));
#8702=CARTESIAN_POINT('Ctrl Pts',(2.99347740802958,0.198964922639276,1.245411532046));
#8703=CARTESIAN_POINT('Ctrl Pts',(2.99609686518216,0.154588504271054,1.20103511367778));
#8704=CARTESIAN_POINT('Ctrl Pts',(2.99749070376198,0.126486346986081,1.18179746841036));
#8705=CARTESIAN_POINT('Ctrl Pts',(2.99945625936844,0.0648957875009219,1.15627950921557));
#8706=CARTESIAN_POINT('Ctrl Pts',(3.,0.0314061622633416,1.15));
#8707=CARTESIAN_POINT('Ctrl Pts',(3.,-0.0314061622633416,1.15));
#8708=CARTESIAN_POINT('Ctrl Pts',(2.99945625936844,-0.0648957875009221,
1.15627950921557));
#8709=CARTESIAN_POINT('Ctrl Pts',(2.99749070376198,-0.126486346986081,1.18179746841036));
#8710=CARTESIAN_POINT('Ctrl Pts',(2.99609686518216,-0.154588504271054,1.20103511367778));
#8711=CARTESIAN_POINT('Ctrl Pts',(2.99347740802958,-0.198964922639276,1.245411532046));
#8712=CARTESIAN_POINT('Ctrl Pts',(2.99208145165098,-0.218202539734559,1.27351367328886));
#8713=CARTESIAN_POINT('Ctrl Pts',(2.99011104995181,-0.24372047740942,1.33510417960069));
#8714=CARTESIAN_POINT('Ctrl Pts',(2.98956518577535,-0.25,1.36859378633186));
#8715=CARTESIAN_POINT('Ctrl Pts',(2.98956518577535,-0.25,1.43140621366814));
#8716=CARTESIAN_POINT('Ctrl Pts',(2.99011104995181,-0.24372047740942,1.4648958203993));
#8717=CARTESIAN_POINT('Ctrl Pts',(2.99208145165098,-0.21820253973456,1.52648632671114));
#8718=CARTESIAN_POINT('Ctrl Pts',(2.99347740802958,-0.198964922639276,1.554588467954));
#8719=CARTESIAN_POINT('Ctrl Pts',(2.99609686518216,-0.154588504271054,1.59896488632222));
#8720=CARTESIAN_POINT('Ctrl Pts',(2.99749070376198,-0.126486346986082,1.61820253158964));
#8721=CARTESIAN_POINT('Ctrl Pts',(2.99945625936844,-0.0648957875009221,
1.64372049078443));
#8722=CARTESIAN_POINT('Ctrl Pts',(3.,-0.0314061622633417,1.65));
#8723=CARTESIAN_POINT('Ctrl Pts',(3.,-5.55111512312578E-17,1.65));
#8724=CARTESIAN_POINT('Ctrl Pts',(3.,-2.08166817117217E-17,1.65));
#8725=CARTESIAN_POINT('Ctrl Pts',(3.,0.0314061622633416,1.65));
#8726=CARTESIAN_POINT('Ctrl Pts',(2.99945625936844,0.0648957875009221,1.64372049078443));
#8727=CARTESIAN_POINT('Ctrl Pts',(2.99749070376198,0.126486346986081,1.61820253158964));
#8728=CARTESIAN_POINT('Ctrl Pts',(2.99609686518216,0.154588504271054,1.59896488632222));
#8729=CARTESIAN_POINT('Ctrl Pts',(2.99347740802958,0.198964922639276,1.554588467954));
#8730=CARTESIAN_POINT('Ctrl Pts',(2.99208145165098,0.218202539734559,1.52648632671114));
#8731=CARTESIAN_POINT('Ctrl Pts',(2.99011104995181,0.24372047740942,1.46489582039931));
#8732=CARTESIAN_POINT('Ctrl Pts',(2.98956518577535,0.25,1.43140621366814));
#8733=CARTESIAN_POINT('Ctrl Pts',(2.98956518577535,0.25,1.4));
#8734=CARTESIAN_POINT('Origin',(-1.23743686707646,-1.23743686707646,2.9));
#8735=CARTESIAN_POINT('',(-1.40243686707646,-1.23743686707646,2.9));
#8736=CARTESIAN_POINT('Origin',(-1.23743686707646,-1.23743686707646,2.9));
#8737=CARTESIAN_POINT('',(-1.40243686707646,-1.23743686707646,3.6));
#8738=CARTESIAN_POINT('',(-1.40243686707646,-1.23743686707646,2.9));
#8739=CARTESIAN_POINT('Origin',(-1.23743686707646,-1.23743686707646,3.6));
#8740=CARTESIAN_POINT('Origin',(-1.23743686707646,-1.23743686707646,2.9));
#8741=CARTESIAN_POINT('Origin',(-1.23743686707646,1.23743686707646,2.9));
#8742=CARTESIAN_POINT('',(-1.40243686707646,1.23743686707646,2.9));
#8743=CARTESIAN_POINT('Origin',(-1.23743686707646,1.23743686707646,2.9));
#8744=CARTESIAN_POINT('',(-1.40243686707646,1.23743686707646,3.6));
#8745=CARTESIAN_POINT('',(-1.40243686707646,1.23743686707646,2.9));
#8746=CARTESIAN_POINT('Origin',(-1.23743686707646,1.23743686707646,3.6));
#8747=CARTESIAN_POINT('Origin',(-1.23743686707646,1.23743686707646,2.9));
#8748=CARTESIAN_POINT('Origin',(1.23743686707646,1.23743686707646,2.9));
#8749=CARTESIAN_POINT('',(1.07243686707646,1.23743686707646,2.9));
#8750=CARTESIAN_POINT('Origin',(1.23743686707646,1.23743686707646,2.9));
#8751=CARTESIAN_POINT('',(1.07243686707646,1.23743686707646,3.6));
#8752=CARTESIAN_POINT('',(1.07243686707646,1.23743686707646,2.9));
#8753=CARTESIAN_POINT('Origin',(1.23743686707646,1.23743686707646,3.6));
#8754=CARTESIAN_POINT('Origin',(1.23743686707646,1.23743686707646,2.9));
#8755=CARTESIAN_POINT('Origin',(1.23743686707646,-1.23743686707646,2.9));
#8756=CARTESIAN_POINT('',(1.07243686707646,-1.23743686707646,2.9));
#8757=CARTESIAN_POINT('Origin',(1.23743686707646,-1.23743686707646,2.9));
#8758=CARTESIAN_POINT('',(1.07243686707646,-1.23743686707646,3.6));
#8759=CARTESIAN_POINT('',(1.07243686707646,-1.23743686707646,2.9));
#8760=CARTESIAN_POINT('Origin',(1.23743686707646,-1.23743686707646,3.6));
#8761=CARTESIAN_POINT('Origin',(1.23743686707646,-1.23743686707646,2.9));
#8762=CARTESIAN_POINT('Origin',(-1.76776695296637,-1.76776695296637,2.4));
#8763=CARTESIAN_POINT('',(-1.8139637388702,-1.24480341984751,2.4));
#8764=CARTESIAN_POINT('',(-1.24480341984751,-1.81396373887019,2.4));
#8765=CARTESIAN_POINT('Origin',(0.,0.,2.4));
#8766=CARTESIAN_POINT('Origin',(-1.76776695296637,-1.76776695296637,2.4));
#8767=CARTESIAN_POINT('Origin',(-1.76776695296637,-1.76776695296637,1.8));
#8768=CARTESIAN_POINT('',(-1.8139637388702,-1.24480341984751,1.8));
#8769=CARTESIAN_POINT('',(-1.8139637388702,-1.24480341984751,1.8));
#8770=CARTESIAN_POINT('',(-1.24480341984751,-1.81396373887019,1.8));
#8771=CARTESIAN_POINT('Origin',(-1.76776695296637,-1.76776695296637,1.8));
#8772=CARTESIAN_POINT('',(-1.24480341984751,-1.81396373887019,1.8));
#8773=CARTESIAN_POINT('Origin',(-1.76776695296637,1.76776695296637,1.8));
#8774=CARTESIAN_POINT('',(-1.81396373887019,1.24480341984751,2.4));
#8775=CARTESIAN_POINT('',(-1.81396373887019,1.24480341984751,1.8));
#8776=CARTESIAN_POINT('',(-1.81396373887019,1.24480341984751,1.8));
#8777=CARTESIAN_POINT('',(-1.24480341984751,1.81396373887019,2.4));
#8778=CARTESIAN_POINT('Origin',(-1.76776695296637,1.76776695296637,2.4));
#8779=CARTESIAN_POINT('',(-1.24480341984751,1.81396373887019,1.8));
#8780=CARTESIAN_POINT('',(-1.24480341984751,1.81396373887019,1.8));
#8781=CARTESIAN_POINT('Origin',(-1.76776695296637,1.76776695296637,1.8));
#8782=CARTESIAN_POINT('Origin',(-1.76776695296637,1.76776695296637,2.4));
#8783=CARTESIAN_POINT('Origin',(0.,0.,2.4));
#8784=CARTESIAN_POINT('Origin',(1.76776695296637,1.76776695296637,1.8));
#8785=CARTESIAN_POINT('',(1.24480341984751,1.81396373887019,2.4));
#8786=CARTESIAN_POINT('',(1.24480341984751,1.81396373887019,1.8));
#8787=CARTESIAN_POINT('',(1.24480341984751,1.81396373887019,1.8));
#8788=CARTESIAN_POINT('',(1.81396373887019,1.24480341984751,2.4));
#8789=CARTESIAN_POINT('Origin',(1.76776695296637,1.76776695296637,2.4));
#8790=CARTESIAN_POINT('',(1.81396373887019,1.24480341984751,1.8));
#8791=CARTESIAN_POINT('',(1.81396373887019,1.24480341984751,1.8));
#8792=CARTESIAN_POINT('Origin',(1.76776695296637,1.76776695296637,1.8));
#8793=CARTESIAN_POINT('Origin',(1.76776695296637,1.76776695296637,2.4));
#8794=CARTESIAN_POINT('Origin',(0.,0.,2.4));
#8795=CARTESIAN_POINT('Origin',(1.76776695296637,-1.76776695296637,1.8));
#8796=CARTESIAN_POINT('',(1.81396373887019,-1.24480341984751,2.4));
#8797=CARTESIAN_POINT('',(1.81396373887019,-1.24480341984751,1.8));
#8798=CARTESIAN_POINT('',(1.81396373887019,-1.24480341984751,1.8));
#8799=CARTESIAN_POINT('',(1.24480341984751,-1.8139637388702,2.4));
#8800=CARTESIAN_POINT('Origin',(1.76776695296637,-1.76776695296637,2.4));
#8801=CARTESIAN_POINT('',(1.24480341984751,-1.8139637388702,1.8));
#8802=CARTESIAN_POINT('',(1.24480341984751,-1.8139637388702,1.8));
#8803=CARTESIAN_POINT('Origin',(1.76776695296637,-1.76776695296637,1.8));
#8804=CARTESIAN_POINT('Origin',(1.76776695296637,-1.76776695296637,2.4));
#8805=CARTESIAN_POINT('Origin',(0.,0.,2.4));
#8806=CARTESIAN_POINT('Origin',(0.,0.,1.));
#8807=CARTESIAN_POINT('',(-2.2,-2.69422295812418E-16,3.6));
#8808=CARTESIAN_POINT('Origin',(0.,0.,3.6));
#8809=CARTESIAN_POINT('',(-2.2,-2.69422295812418E-16,1.8));
#8810=CARTESIAN_POINT('',(-2.2,-2.69422295812418E-16,1.));
#8811=CARTESIAN_POINT('Origin',(0.,0.,1.8));
#8812=CARTESIAN_POINT('Origin',(0.,0.,1.8));
#8813=CARTESIAN_POINT('Origin',(0.,0.,1.8));
#8814=CARTESIAN_POINT('Origin',(0.,0.,1.8));
#8815=CARTESIAN_POINT('Origin',(0.,0.,1.8));
#8816=CARTESIAN_POINT('Origin',(0.,0.,1.8));
#8817=CARTESIAN_POINT('',(-3.,-3.67394039744206E-16,1.8));
#8818=CARTESIAN_POINT('Origin',(0.,0.,1.8));
#8819=CARTESIAN_POINT('',(-2.04276695296637,-1.76776695296637,1.8));
#8820=CARTESIAN_POINT('Origin',(-1.76776695296637,-1.76776695296637,1.8));
#8821=CARTESIAN_POINT('',(1.49276695296637,1.76776695296637,1.8));
#8822=CARTESIAN_POINT('Origin',(1.76776695296637,1.76776695296637,1.8));
#8823=CARTESIAN_POINT('',(1.49276695296637,-1.76776695296637,1.8));
#8824=CARTESIAN_POINT('Origin',(1.76776695296637,-1.76776695296637,1.8));
#8825=CARTESIAN_POINT('',(-2.04276695296637,1.76776695296637,1.8));
#8826=CARTESIAN_POINT('Origin',(-1.76776695296637,1.76776695296637,1.8));
#8827=CARTESIAN_POINT('Origin',(-1.76776695296637,-1.76776695296637,0.9));
#8828=CARTESIAN_POINT('',(-2.04276695296637,-1.76776695296637,1.));
#8829=CARTESIAN_POINT('Origin',(-1.76776695296637,-1.76776695296637,1.));
#8830=CARTESIAN_POINT('',(-2.04276695296637,-1.76776695296637,0.9));
#8831=CARTESIAN_POINT('Origin',(-1.76776695296637,1.76776695296637,0.9));
#8832=CARTESIAN_POINT('',(-2.04276695296637,1.76776695296637,1.));
#8833=CARTESIAN_POINT('Origin',(-1.76776695296637,1.76776695296637,1.));
#8834=CARTESIAN_POINT('',(-2.04276695296637,1.76776695296637,0.9));
#8835=CARTESIAN_POINT('Origin',(1.76776695296637,1.76776695296637,0.9));
#8836=CARTESIAN_POINT('',(1.49276695296637,1.76776695296637,1.));
#8837=CARTESIAN_POINT('Origin',(1.76776695296637,1.76776695296637,1.));
#8838=CARTESIAN_POINT('',(1.49276695296637,1.76776695296637,0.9));
#8839=CARTESIAN_POINT('Origin',(1.76776695296637,-1.76776695296637,0.9));
#8840=CARTESIAN_POINT('',(1.49276695296637,-1.76776695296637,1.));
#8841=CARTESIAN_POINT('Origin',(1.76776695296637,-1.76776695296637,1.));
#8842=CARTESIAN_POINT('',(1.49276695296637,-1.76776695296637,0.9));
#8843=CARTESIAN_POINT('Origin',(0.,0.,2.05));
#8844=CARTESIAN_POINT('',(-1.5,-1.83697019872103E-16,2.05));
#8845=CARTESIAN_POINT('Origin',(0.,0.,2.05));
#8846=CARTESIAN_POINT('',(-1.5,1.83697019872103E-16,3.6));
#8847=CARTESIAN_POINT('',(-1.5,-1.83697019872103E-16,2.05));
#8848=CARTESIAN_POINT('Origin',(0.,0.,3.6));
#8849=CARTESIAN_POINT('Origin',(0.,0.,2.05));
#8850=CARTESIAN_POINT('',(-1.02,-1.2491397351303E-16,2.05));
#8851=CARTESIAN_POINT('Origin',(0.,0.,2.05));
#8852=CARTESIAN_POINT('Origin',(0.,0.,1.));
#8853=CARTESIAN_POINT('',(-3.,-3.67394039744206E-16,1.));
#8854=CARTESIAN_POINT('',(-3.,-3.67394039744206E-16,1.));
#8855=CARTESIAN_POINT('Origin',(0.,0.,1.));
#8856=CARTESIAN_POINT('Origin',(0.,0.,1.));
#8857=CARTESIAN_POINT('',(-1.02,-1.2491397351303E-16,1.));
#8858=CARTESIAN_POINT('',(-1.02,-1.2491397351303E-16,1.));
#8859=CARTESIAN_POINT('Origin',(0.,0.,1.));
#8860=CARTESIAN_POINT('Origin',(0.,0.,3.6));
#8861=CARTESIAN_POINT('Origin',(0.,0.,1.));
#10577=UNCERTAINTY_MEASURE_WITH_UNIT(LENGTH_MEASURE(0.001),#10651,
'DISTANCE_ACCURACY_VALUE',
'Maximum model space distance between geometric entities at asserted c
onnectivities');
#10611=UNCERTAINTY_MEASURE_WITH_UNIT(LENGTH_MEASURE(0.001),#10651,
'DISTANCE_ACCURACY_VALUE',
'Maximum model space distance between geometric entities at asserted c
onnectivities');
#10616=(
GEOMETRIC_REPRESENTATION_CONTEXT(3)
GLOBAL_UNCERTAINTY_ASSIGNED_CONTEXT((#10577))
GLOBAL_UNIT_ASSIGNED_CONTEXT((#10651,#10653,#10654))
REPRESENTATION_CONTEXT('','3D')
);
#10650=(
GEOMETRIC_REPRESENTATION_CONTEXT(3)
GLOBAL_UNCERTAINTY_ASSIGNED_CONTEXT((#10611))
GLOBAL_UNIT_ASSIGNED_CONTEXT((#10651,#10653,#10654))
REPRESENTATION_CONTEXT('','3D')
);
#10651=(
LENGTH_UNIT()
NAMED_UNIT(*)
SI_UNIT(.CENTI.,.METRE.)
);
#10653=(
NAMED_UNIT(*)
PLANE_ANGLE_UNIT()
SI_UNIT($,.RADIAN.)
);
#10654=(
NAMED_UNIT(*)
SI_UNIT($,.STERADIAN.)
SOLID_ANGLE_UNIT()
);
#10659=SHAPE_DEFINITION_REPRESENTATION(#10697,#10798);
#10697=PRODUCT_DEFINITION_SHAPE('',$,#10837);
#10798=SHAPE_REPRESENTATION('',(#5972),#10616);
#10832=PRODUCT_DEFINITION_CONTEXT('part definition',#10948,'design');
#10837=PRODUCT_DEFINITION('Pivot pedestal','Pivot pedestal',#10875,#10832);
#10875=PRODUCT_DEFINITION_FORMATION('',$,#10954);
#10948=APPLICATION_CONTEXT(
'Core Data for Automotive Mechanical Design Process');
#10949=PRODUCT_CONTEXT('part definition',#10948,'mechanical');
#10954=PRODUCT('Pivot pedestal','Pivot pedestal','Pivot pedestal',(#10949));
#11072=COLOUR_RGB('Off White',0.89,0.88,0.83);
#11073=FILL_AREA_STYLE_COLOUR('',#11072);
#11074=FILL_AREA_STYLE('',(#11073));
#11075=SURFACE_STYLE_FILL_AREA(#11074);
#11076=SURFACE_SIDE_STYLE('',(#11075));
#11077=SURFACE_STYLE_USAGE(.BOTH.,#11076);
#11078=PRESENTATION_STYLE_ASSIGNMENT((#11077));
ENDSEC;
END-ISO-10303-21;
